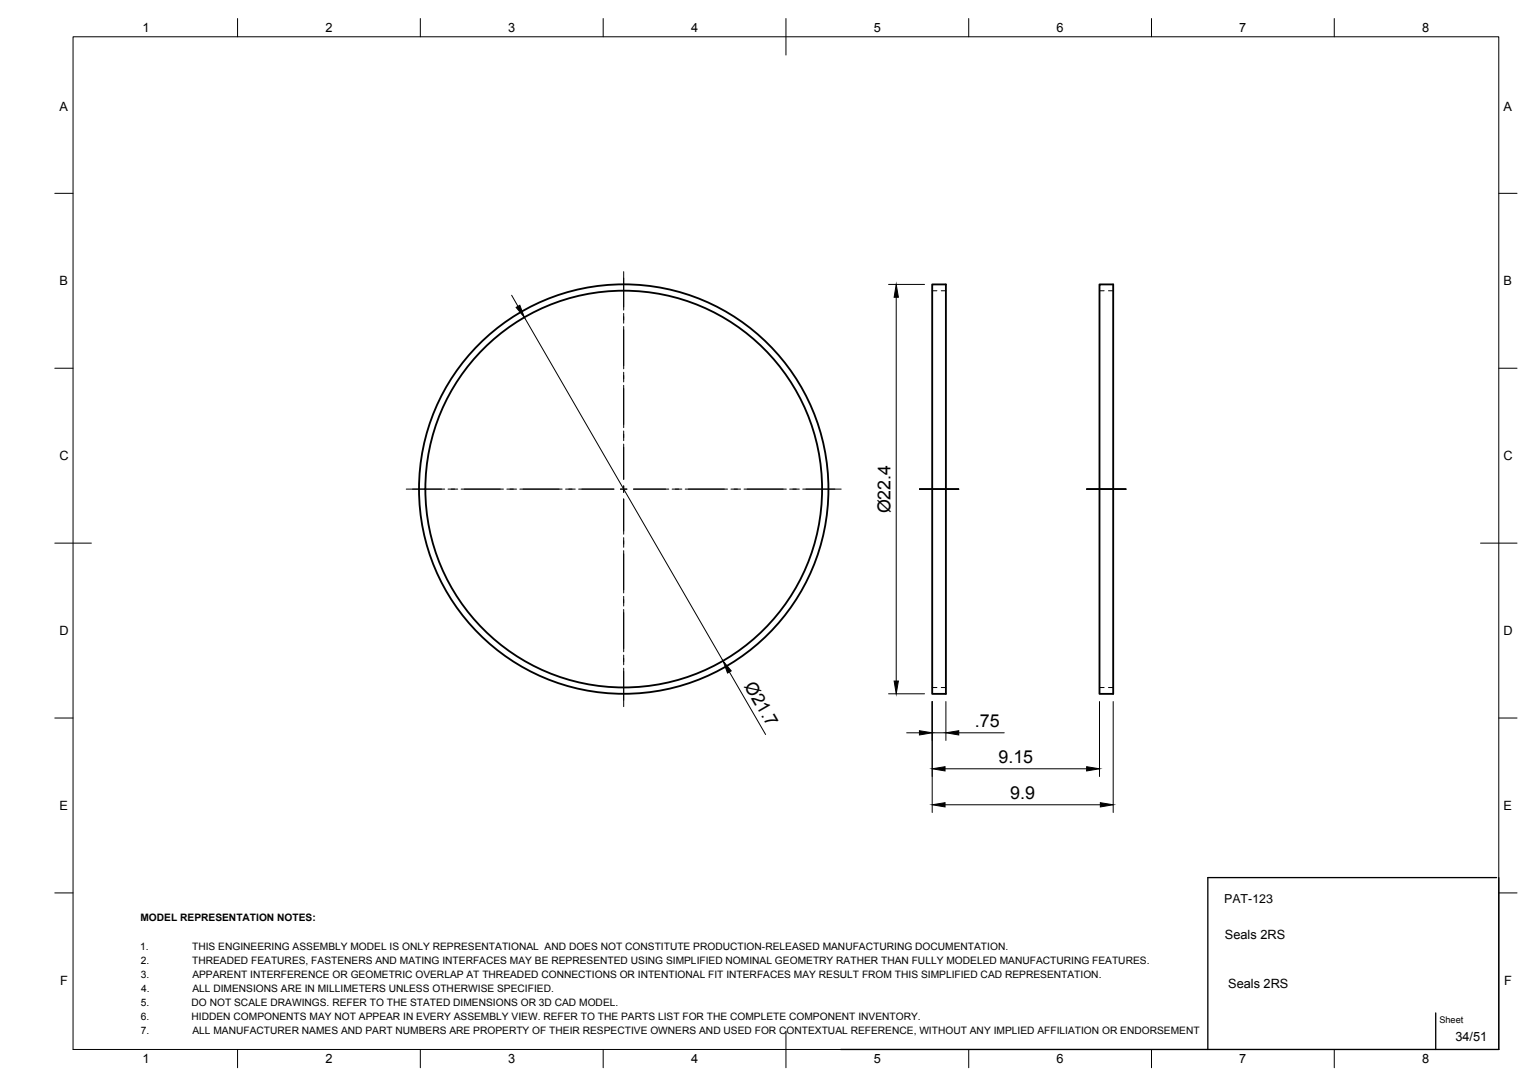
ISO-10303-21;
HEADER;
/* Generated by software containing ST-Developer
 * from STEP Tools, Inc. (www.steptools.com) 
 */

FILE_DESCRIPTION(
/* description */ ('Worm-less right-angle friction wheel drive'),
/* implementation_level */ '2;1');

FILE_NAME(
/* name */ 'Seals 2RS.step',
/* time_stamp */ '2026-10-28T03:22:36-07:00',
/* author */ (''),
/* organization */ (''),
/* preprocessor_version */ 'ST-DEVELOPER v20.2',
/* originating_system */ 'Autodesk Translation Framework v15.17.0.0',
/* authorisation */ '');

FILE_SCHEMA (('AUTOMOTIVE_DESIGN { 1 0 10303 214 3 1 1 }'));
ENDSEC;

DATA;
#10=MECHANICAL_DESIGN_GEOMETRIC_PRESENTATION_REPRESENTATION('',(#645,#646),#17046);
#545=SHAPE_REPRESENTATION_RELATIONSHIP('SRR','None',#17289,#592);
#592=ADVANCED_BREP_SHAPE_REPRESENTATION('',(#698,#699),#17025);
#645=STYLED_ITEM('',(#17591),#698);
#646=STYLED_ITEM('',(#17591),#699);
#698=MANIFOLD_SOLID_BREP('Body1',#8201);
#699=MANIFOLD_SOLID_BREP('Body2',#8202);
#911=FACE_BOUND('',#2162,.T.);
#912=FACE_BOUND('',#2165,.T.);
#913=FACE_BOUND('',#2168,.T.);
#914=FACE_BOUND('',#2171,.T.);
#1091=PLANE('',#9368);
#1092=PLANE('',#9373);
#1093=PLANE('',#9376);
#1094=PLANE('',#9381);
#1499=FACE_OUTER_BOUND('',#2161,.T.);
#1500=FACE_OUTER_BOUND('',#2163,.T.);
#1501=FACE_OUTER_BOUND('',#2164,.T.);
#1502=FACE_OUTER_BOUND('',#2166,.T.);
#1503=FACE_OUTER_BOUND('',#2167,.T.);
#1504=FACE_OUTER_BOUND('',#2169,.T.);
#1505=FACE_OUTER_BOUND('',#2170,.T.);
#1506=FACE_OUTER_BOUND('',#2172,.T.);
#2161=EDGE_LOOP('',(#6840));
#2162=EDGE_LOOP('',(#6841));
#2163=EDGE_LOOP('',(#6842,#6843,#6844,#6845));
#2164=EDGE_LOOP('',(#6846));
#2165=EDGE_LOOP('',(#6847));
#2166=EDGE_LOOP('',(#6848,#6849,#6850,#6851));
#2167=EDGE_LOOP('',(#6852));
#2168=EDGE_LOOP('',(#6853));
#2169=EDGE_LOOP('',(#6854,#6855,#6856,#6857));
#2170=EDGE_LOOP('',(#6858));
#2171=EDGE_LOOP('',(#6859));
#2172=EDGE_LOOP('',(#6860,#6861,#6862,#6863));
#2709=LINE('',#15895,#3249);
#2710=LINE('',#15900,#3250);
#2711=LINE('',#15909,#3251);
#2712=LINE('',#15914,#3252);
#3249=VECTOR('',#11367,1.119765);
#3250=VECTOR('',#11374,1.085235);
#3251=VECTOR('',#11385,1.119765);
#3252=VECTOR('',#11392,1.085235);
#3762=CIRCLE('',#9369,1.119765);
#3763=CIRCLE('',#9370,1.085235);
#3764=CIRCLE('',#9372,1.119765);
#3765=CIRCLE('',#9374,1.085235);
#3766=CIRCLE('',#9377,1.119765);
#3767=CIRCLE('',#9378,1.085235);
#3768=CIRCLE('',#9380,1.119765);
#3769=CIRCLE('',#9382,1.085235);
#4311=VERTEX_POINT('',#15888);
#4312=VERTEX_POINT('',#15890);
#4313=VERTEX_POINT('',#15893);
#4314=VERTEX_POINT('',#15897);
#4315=VERTEX_POINT('',#15902);
#4316=VERTEX_POINT('',#15904);
#4317=VERTEX_POINT('',#15907);
#4318=VERTEX_POINT('',#15911);
#5189=EDGE_CURVE('',#4311,#4311,#3762,.T.);
#5190=EDGE_CURVE('',#4312,#4312,#3763,.T.);
#5191=EDGE_CURVE('',#4313,#4313,#3764,.T.);
#5192=EDGE_CURVE('',#4313,#4311,#2709,.T.);
#5193=EDGE_CURVE('',#4314,#4314,#3765,.T.);
#5194=EDGE_CURVE('',#4314,#4312,#2710,.T.);
#5195=EDGE_CURVE('',#4315,#4315,#3766,.T.);
#5196=EDGE_CURVE('',#4316,#4316,#3767,.T.);
#5197=EDGE_CURVE('',#4317,#4317,#3768,.T.);
#5198=EDGE_CURVE('',#4317,#4315,#2711,.T.);
#5199=EDGE_CURVE('',#4318,#4318,#3769,.T.);
#5200=EDGE_CURVE('',#4318,#4316,#2712,.T.);
#6840=ORIENTED_EDGE('',*,*,#5189,.F.);
#6841=ORIENTED_EDGE('',*,*,#5190,.T.);
#6842=ORIENTED_EDGE('',*,*,#5191,.F.);
#6843=ORIENTED_EDGE('',*,*,#5192,.T.);
#6844=ORIENTED_EDGE('',*,*,#5189,.T.);
#6845=ORIENTED_EDGE('',*,*,#5192,.F.);
#6846=ORIENTED_EDGE('',*,*,#5191,.T.);
#6847=ORIENTED_EDGE('',*,*,#5193,.F.);
#6848=ORIENTED_EDGE('',*,*,#5193,.T.);
#6849=ORIENTED_EDGE('',*,*,#5194,.T.);
#6850=ORIENTED_EDGE('',*,*,#5190,.F.);
#6851=ORIENTED_EDGE('',*,*,#5194,.F.);
#6852=ORIENTED_EDGE('',*,*,#5195,.F.);
#6853=ORIENTED_EDGE('',*,*,#5196,.T.);
#6854=ORIENTED_EDGE('',*,*,#5197,.F.);
#6855=ORIENTED_EDGE('',*,*,#5198,.T.);
#6856=ORIENTED_EDGE('',*,*,#5195,.T.);
#6857=ORIENTED_EDGE('',*,*,#5198,.F.);
#6858=ORIENTED_EDGE('',*,*,#5197,.T.);
#6859=ORIENTED_EDGE('',*,*,#5199,.F.);
#6860=ORIENTED_EDGE('',*,*,#5199,.T.);
#6861=ORIENTED_EDGE('',*,*,#5200,.T.);
#6862=ORIENTED_EDGE('',*,*,#5196,.F.);
#6863=ORIENTED_EDGE('',*,*,#5200,.F.);
#7656=CYLINDRICAL_SURFACE('',#9371,1.119765);
#7657=CYLINDRICAL_SURFACE('',#9375,1.085235);
#7658=CYLINDRICAL_SURFACE('',#9379,1.119765);
#7659=CYLINDRICAL_SURFACE('',#9383,1.085235);
#7991=ADVANCED_FACE('',(#1499,#911),#1091,.T.);
#7992=ADVANCED_FACE('',(#1500),#7656,.T.);
#7993=ADVANCED_FACE('',(#1501,#912),#1092,.T.);
#7994=ADVANCED_FACE('',(#1502),#7657,.F.);
#7995=ADVANCED_FACE('',(#1503,#913),#1093,.T.);
#7996=ADVANCED_FACE('',(#1504),#7658,.T.);
#7997=ADVANCED_FACE('',(#1505,#914),#1094,.T.);
#7998=ADVANCED_FACE('',(#1506),#7659,.F.);
#8201=CLOSED_SHELL('',(#7991,#7992,#7993,#7994));
#8202=CLOSED_SHELL('',(#7995,#7996,#7997,#7998));
#9367=AXIS2_PLACEMENT_3D('',#15886,#11355,#11356);
#9368=AXIS2_PLACEMENT_3D('',#15887,#11357,#11358);
#9369=AXIS2_PLACEMENT_3D('',#15889,#11359,#11360);
#9370=AXIS2_PLACEMENT_3D('',#15891,#11361,#11362);
#9371=AXIS2_PLACEMENT_3D('',#15892,#11363,#11364);
#9372=AXIS2_PLACEMENT_3D('',#15894,#11365,#11366);
#9373=AXIS2_PLACEMENT_3D('',#15896,#11368,#11369);
#9374=AXIS2_PLACEMENT_3D('',#15898,#11370,#11371);
#9375=AXIS2_PLACEMENT_3D('',#15899,#11372,#11373);
#9376=AXIS2_PLACEMENT_3D('',#15901,#11375,#11376);
#9377=AXIS2_PLACEMENT_3D('',#15903,#11377,#11378);
#9378=AXIS2_PLACEMENT_3D('',#15905,#11379,#11380);
#9379=AXIS2_PLACEMENT_3D('',#15906,#11381,#11382);
#9380=AXIS2_PLACEMENT_3D('',#15908,#11383,#11384);
#9381=AXIS2_PLACEMENT_3D('',#15910,#11386,#11387);
#9382=AXIS2_PLACEMENT_3D('',#15912,#11388,#11389);
#9383=AXIS2_PLACEMENT_3D('',#15913,#11390,#11391);
#11355=DIRECTION('axis',(0.,0.,1.));
#11356=DIRECTION('refdir',(1.,0.,0.));
#11357=DIRECTION('center_axis',(0.,1.,0.));
#11358=DIRECTION('ref_axis',(0.,0.,1.));
#11359=DIRECTION('center_axis',(0.,-1.,0.));
#11360=DIRECTION('ref_axis',(1.,0.,0.));
#11361=DIRECTION('center_axis',(0.,-1.,0.));
#11362=DIRECTION('ref_axis',(1.,0.,0.));
#11363=DIRECTION('center_axis',(0.,-1.,0.));
#11364=DIRECTION('ref_axis',(1.,0.,0.));
#11365=DIRECTION('center_axis',(0.,-1.,0.));
#11366=DIRECTION('ref_axis',(1.,0.,0.));
#11367=DIRECTION('',(0.,1.,0.));
#11368=DIRECTION('center_axis',(0.,-1.,0.));
#11369=DIRECTION('ref_axis',(0.,0.,-1.));
#11370=DIRECTION('center_axis',(0.,-1.,0.));
#11371=DIRECTION('ref_axis',(1.,0.,0.));
#11372=DIRECTION('center_axis',(0.,-1.,0.));
#11373=DIRECTION('ref_axis',(1.,0.,0.));
#11374=DIRECTION('',(0.,1.,0.));
#11375=DIRECTION('center_axis',(0.,1.,0.));
#11376=DIRECTION('ref_axis',(0.,0.,1.));
#11377=DIRECTION('center_axis',(0.,-1.,0.));
#11378=DIRECTION('ref_axis',(1.,0.,0.));
#11379=DIRECTION('center_axis',(0.,-1.,0.));
#11380=DIRECTION('ref_axis',(1.,0.,0.));
#11381=DIRECTION('center_axis',(0.,-1.,0.));
#11382=DIRECTION('ref_axis',(1.,0.,0.));
#11383=DIRECTION('center_axis',(0.,-1.,0.));
#11384=DIRECTION('ref_axis',(1.,0.,0.));
#11385=DIRECTION('',(0.,1.,0.));
#11386=DIRECTION('center_axis',(0.,-1.,0.));
#11387=DIRECTION('ref_axis',(0.,0.,-1.));
#11388=DIRECTION('center_axis',(0.,-1.,0.));
#11389=DIRECTION('ref_axis',(1.,0.,0.));
#11390=DIRECTION('center_axis',(0.,-1.,0.));
#11391=DIRECTION('ref_axis',(1.,0.,0.));
#11392=DIRECTION('',(0.,1.,0.));
#15886=CARTESIAN_POINT('',(0.,0.,0.));
#15887=CARTESIAN_POINT('Origin',(1.119765,0.495,0.));
#15888=CARTESIAN_POINT('',(-1.119765,0.495,-1.37131662304724E-16));
#15889=CARTESIAN_POINT('Origin',(0.,0.495,0.));
#15890=CARTESIAN_POINT('',(-1.085235,0.495,-1.32902956907268E-16));
#15891=CARTESIAN_POINT('Origin',(0.,0.495,0.));
#15892=CARTESIAN_POINT('Origin',(0.,0.4575,0.));
#15893=CARTESIAN_POINT('',(-1.119765,0.42,-1.37131662304724E-16));
#15894=CARTESIAN_POINT('Origin',(0.,0.42,0.));
#15895=CARTESIAN_POINT('',(-1.119765,0.4575,-1.37131662304724E-16));
#15896=CARTESIAN_POINT('Origin',(1.085235,0.42,0.));
#15897=CARTESIAN_POINT('',(-1.085235,0.42,-1.32902956907268E-16));
#15898=CARTESIAN_POINT('Origin',(0.,0.42,0.));
#15899=CARTESIAN_POINT('Origin',(0.,0.4575,0.));
#15900=CARTESIAN_POINT('',(-1.085235,0.4575,-1.32902956907268E-16));
#15901=CARTESIAN_POINT('Origin',(1.119765,-0.42,0.));
#15902=CARTESIAN_POINT('',(-1.119765,-0.42,-1.37131662304724E-16));
#15903=CARTESIAN_POINT('Origin',(0.,-0.42,0.));
#15904=CARTESIAN_POINT('',(-1.085235,-0.42,-1.32902956907268E-16));
#15905=CARTESIAN_POINT('Origin',(0.,-0.42,0.));
#15906=CARTESIAN_POINT('Origin',(0.,-0.4575,0.));
#15907=CARTESIAN_POINT('',(-1.119765,-0.495,-1.37131662304724E-16));
#15908=CARTESIAN_POINT('Origin',(0.,-0.495,0.));
#15909=CARTESIAN_POINT('',(-1.119765,-0.4575,-1.37131662304724E-16));
#15910=CARTESIAN_POINT('Origin',(1.085235,-0.495,0.));
#15911=CARTESIAN_POINT('',(-1.085235,-0.495,-1.32902956907268E-16));
#15912=CARTESIAN_POINT('Origin',(0.,-0.495,0.));
#15913=CARTESIAN_POINT('Origin',(0.,-0.4575,0.));
#15914=CARTESIAN_POINT('',(-1.085235,-0.4575,-1.32902956907268E-16));
#16972=UNCERTAINTY_MEASURE_WITH_UNIT(LENGTH_MEASURE(0.001),#17047,
'DISTANCE_ACCURACY_VALUE',
'Maximum model space distance between geometric entities at asserted c
onnectivities');
#16993=UNCERTAINTY_MEASURE_WITH_UNIT(LENGTH_MEASURE(0.001),#17047,
'DISTANCE_ACCURACY_VALUE',
'Maximum model space distance between geometric entities at asserted c
onnectivities');
#17025=(
GEOMETRIC_REPRESENTATION_CONTEXT(3)
GLOBAL_UNCERTAINTY_ASSIGNED_CONTEXT((#16972))
GLOBAL_UNIT_ASSIGNED_CONTEXT((#17047,#17049,#17050))
REPRESENTATION_CONTEXT('','3D')
);
#17046=(
GEOMETRIC_REPRESENTATION_CONTEXT(3)
GLOBAL_UNCERTAINTY_ASSIGNED_CONTEXT((#16993))
GLOBAL_UNIT_ASSIGNED_CONTEXT((#17047,#17049,#17050))
REPRESENTATION_CONTEXT('','3D')
);
#17047=(
LENGTH_UNIT()
NAMED_UNIT(*)
SI_UNIT(.CENTI.,.METRE.)
);
#17049=(
NAMED_UNIT(*)
PLANE_ANGLE_UNIT()
SI_UNIT($,.RADIAN.)
);
#17050=(
NAMED_UNIT(*)
SI_UNIT($,.STERADIAN.)
SOLID_ANGLE_UNIT()
);
#17082=SHAPE_DEFINITION_REPRESENTATION(#17134,#17289);
#17134=PRODUCT_DEFINITION_SHAPE('',$,#17342);
#17289=SHAPE_REPRESENTATION('',(#9367),#17025);
#17310=PRODUCT_DEFINITION_CONTEXT('part definition',#17468,'design');
#17342=PRODUCT_DEFINITION('Seals 2RS','Seals 2RS',#17394,#17310);
#17394=PRODUCT_DEFINITION_FORMATION('',$,#17501);
#17468=APPLICATION_CONTEXT(
'Core Data for Automotive Mechanical Design Process');
#17469=PRODUCT_CONTEXT('part definition',#17468,'mechanical');
#17501=PRODUCT('Seals 2RS','Seals 2RS','Seals 2RS',(#17469));
#17585=COLOUR_RGB('Grey',0.48,0.52,0.57);
#17586=FILL_AREA_STYLE_COLOUR('',#17585);
#17587=FILL_AREA_STYLE('',(#17586));
#17588=SURFACE_STYLE_FILL_AREA(#17587);
#17589=SURFACE_SIDE_STYLE('',(#17588));
#17590=SURFACE_STYLE_USAGE(.BOTH.,#17589);
#17591=PRESENTATION_STYLE_ASSIGNMENT((#17590));
ENDSEC;
END-ISO-10303-21;
